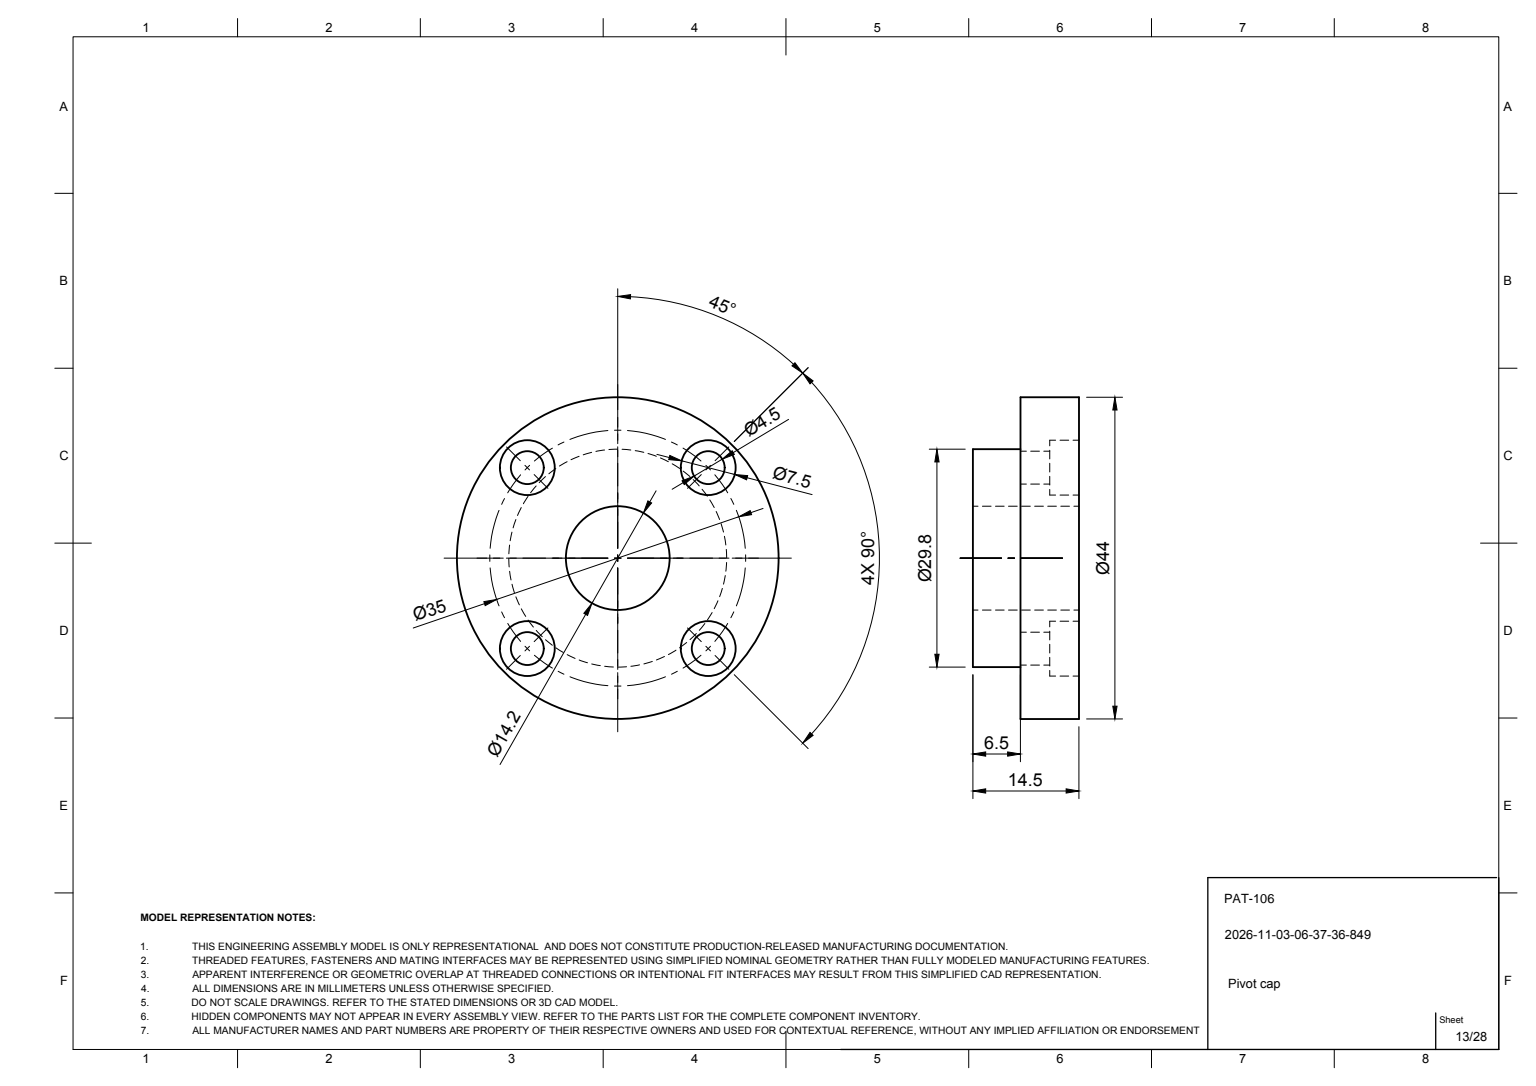
ISO-10303-21;
HEADER;
/* Generated by software containing ST-Developer
 * from STEP Tools, Inc. (www.steptools.com) 
 */

FILE_DESCRIPTION(
/* description */ ('Torsion-spring ratchet demonstrator'),
/* implementation_level */ '2;1');

FILE_NAME(
/* name */ 'Pivot cap.step',
/* time_stamp */ '2026-10-29T17:29:17-07:00',
/* author */ (''),
/* organization */ (''),
/* preprocessor_version */ 'ST-DEVELOPER v20.2',
/* originating_system */ 'Autodesk Translation Framework v15.17.0.0',
/* authorisation */ '');

FILE_SCHEMA (('AUTOMOTIVE_DESIGN { 1 0 10303 214 3 1 1 }'));
ENDSEC;

DATA;
#10=MECHANICAL_DESIGN_GEOMETRIC_PRESENTATION_REPRESENTATION('',(#291),#11258);
#243=SHAPE_REPRESENTATION_RELATIONSHIP('SRR','None',#11369,#267);
#267=ADVANCED_BREP_SHAPE_REPRESENTATION('',(#323),#11239);
#291=STYLED_ITEM('',(#11570),#323);
#323=MANIFOLD_SOLID_BREP('Body1',#5162);
#394=FACE_BOUND('',#1065,.T.);
#395=FACE_BOUND('',#1068,.T.);
#396=FACE_BOUND('',#1071,.T.);
#397=FACE_BOUND('',#1074,.T.);
#398=FACE_BOUND('',#1081,.T.);
#399=FACE_BOUND('',#1085,.T.);
#400=FACE_BOUND('',#1086,.T.);
#401=FACE_BOUND('',#1087,.T.);
#402=FACE_BOUND('',#1088,.T.);
#403=FACE_BOUND('',#1089,.T.);
#404=FACE_BOUND('',#1091,.T.);
#405=FACE_BOUND('',#1092,.T.);
#406=FACE_BOUND('',#1093,.T.);
#407=FACE_BOUND('',#1094,.T.);
#408=FACE_BOUND('',#1095,.T.);
#482=PLANE('',#5643);
#483=PLANE('',#5648);
#484=PLANE('',#5653);
#485=PLANE('',#5658);
#486=PLANE('',#5671);
#487=PLANE('',#5678);
#488=PLANE('',#5679);
#709=FACE_OUTER_BOUND('',#1063,.T.);
#710=FACE_OUTER_BOUND('',#1064,.T.);
#711=FACE_OUTER_BOUND('',#1066,.T.);
#712=FACE_OUTER_BOUND('',#1067,.T.);
#713=FACE_OUTER_BOUND('',#1069,.T.);
#714=FACE_OUTER_BOUND('',#1070,.T.);
#715=FACE_OUTER_BOUND('',#1072,.T.);
#716=FACE_OUTER_BOUND('',#1073,.T.);
#717=FACE_OUTER_BOUND('',#1075,.T.);
#718=FACE_OUTER_BOUND('',#1076,.T.);
#719=FACE_OUTER_BOUND('',#1077,.T.);
#720=FACE_OUTER_BOUND('',#1078,.T.);
#721=FACE_OUTER_BOUND('',#1079,.T.);
#722=FACE_OUTER_BOUND('',#1080,.T.);
#723=FACE_OUTER_BOUND('',#1082,.T.);
#724=FACE_OUTER_BOUND('',#1083,.T.);
#725=FACE_OUTER_BOUND('',#1084,.T.);
#726=FACE_OUTER_BOUND('',#1090,.T.);
#1063=EDGE_LOOP('',(#3796,#3797,#3798,#3799));
#1064=EDGE_LOOP('',(#3800));
#1065=EDGE_LOOP('',(#3801));
#1066=EDGE_LOOP('',(#3802,#3803,#3804,#3805));
#1067=EDGE_LOOP('',(#3806));
#1068=EDGE_LOOP('',(#3807));
#1069=EDGE_LOOP('',(#3808,#3809,#3810,#3811));
#1070=EDGE_LOOP('',(#3812));
#1071=EDGE_LOOP('',(#3813));
#1072=EDGE_LOOP('',(#3814,#3815,#3816,#3817));
#1073=EDGE_LOOP('',(#3818));
#1074=EDGE_LOOP('',(#3819));
#1075=EDGE_LOOP('',(#3820,#3821,#3822,#3823));
#1076=EDGE_LOOP('',(#3824,#3825,#3826,#3827));
#1077=EDGE_LOOP('',(#3828,#3829,#3830,#3831));
#1078=EDGE_LOOP('',(#3832,#3833,#3834,#3835));
#1079=EDGE_LOOP('',(#3836,#3837,#3838,#3839));
#1080=EDGE_LOOP('',(#3840));
#1081=EDGE_LOOP('',(#3841));
#1082=EDGE_LOOP('',(#3842,#3843,#3844,#3845));
#1083=EDGE_LOOP('',(#3846,#3847,#3848,#3849));
#1084=EDGE_LOOP('',(#3850));
#1085=EDGE_LOOP('',(#3851));
#1086=EDGE_LOOP('',(#3852));
#1087=EDGE_LOOP('',(#3853));
#1088=EDGE_LOOP('',(#3854));
#1089=EDGE_LOOP('',(#3855));
#1090=EDGE_LOOP('',(#3856));
#1091=EDGE_LOOP('',(#3857));
#1092=EDGE_LOOP('',(#3858));
#1093=EDGE_LOOP('',(#3859));
#1094=EDGE_LOOP('',(#3860));
#1095=EDGE_LOOP('',(#3861));
#1408=LINE('',#8139,#1791);
#1409=LINE('',#8148,#1792);
#1410=LINE('',#8157,#1793);
#1411=LINE('',#8166,#1794);
#1412=LINE('',#8174,#1795);
#1413=LINE('',#8178,#1796);
#1414=LINE('',#8182,#1797);
#1415=LINE('',#8186,#1798);
#1416=LINE('',#8191,#1799);
#1417=LINE('',#8199,#1800);
#1418=LINE('',#8204,#1801);
#1791=VECTOR('',#6527,0.375);
#1792=VECTOR('',#6538,0.375);
#1793=VECTOR('',#6549,0.375);
#1794=VECTOR('',#6560,0.375);
#1795=VECTOR('',#6571,0.225);
#1796=VECTOR('',#6576,0.225);
#1797=VECTOR('',#6581,0.225);
#1798=VECTOR('',#6586,0.225);
#1799=VECTOR('',#6591,1.49);
#1800=VECTOR('',#6602,0.71);
#1801=VECTOR('',#6607,2.2);
#2181=CIRCLE('',#5641,0.375);
#2182=CIRCLE('',#5642,0.375);
#2183=CIRCLE('',#5644,0.225);
#2184=CIRCLE('',#5646,0.375);
#2185=CIRCLE('',#5647,0.375);
#2186=CIRCLE('',#5649,0.225);
#2187=CIRCLE('',#5651,0.375);
#2188=CIRCLE('',#5652,0.375);
#2189=CIRCLE('',#5654,0.225);
#2190=CIRCLE('',#5656,0.375);
#2191=CIRCLE('',#5657,0.375);
#2192=CIRCLE('',#5659,0.225);
#2193=CIRCLE('',#5661,0.225);
#2194=CIRCLE('',#5663,0.225);
#2195=CIRCLE('',#5665,0.225);
#2196=CIRCLE('',#5667,0.225);
#2197=CIRCLE('',#5669,1.49);
#2198=CIRCLE('',#5670,1.49);
#2199=CIRCLE('',#5672,0.71);
#2200=CIRCLE('',#5674,0.71);
#2201=CIRCLE('',#5676,2.2);
#2202=CIRCLE('',#5677,2.2);
#2453=VERTEX_POINT('',#8136);
#2454=VERTEX_POINT('',#8138);
#2455=VERTEX_POINT('',#8142);
#2456=VERTEX_POINT('',#8145);
#2457=VERTEX_POINT('',#8147);
#2458=VERTEX_POINT('',#8151);
#2459=VERTEX_POINT('',#8154);
#2460=VERTEX_POINT('',#8156);
#2461=VERTEX_POINT('',#8160);
#2462=VERTEX_POINT('',#8163);
#2463=VERTEX_POINT('',#8165);
#2464=VERTEX_POINT('',#8169);
#2465=VERTEX_POINT('',#8172);
#2466=VERTEX_POINT('',#8176);
#2467=VERTEX_POINT('',#8180);
#2468=VERTEX_POINT('',#8184);
#2469=VERTEX_POINT('',#8188);
#2470=VERTEX_POINT('',#8190);
#2471=VERTEX_POINT('',#8194);
#2472=VERTEX_POINT('',#8197);
#2473=VERTEX_POINT('',#8201);
#2474=VERTEX_POINT('',#8203);
#2958=EDGE_CURVE('',#2453,#2453,#2181,.T.);
#2959=EDGE_CURVE('',#2453,#2454,#1408,.T.);
#2960=EDGE_CURVE('',#2454,#2454,#2182,.T.);
#2961=EDGE_CURVE('',#2455,#2455,#2183,.T.);
#2962=EDGE_CURVE('',#2456,#2456,#2184,.T.);
#2963=EDGE_CURVE('',#2456,#2457,#1409,.T.);
#2964=EDGE_CURVE('',#2457,#2457,#2185,.T.);
#2965=EDGE_CURVE('',#2458,#2458,#2186,.T.);
#2966=EDGE_CURVE('',#2459,#2459,#2187,.T.);
#2967=EDGE_CURVE('',#2459,#2460,#1410,.T.);
#2968=EDGE_CURVE('',#2460,#2460,#2188,.T.);
#2969=EDGE_CURVE('',#2461,#2461,#2189,.T.);
#2970=EDGE_CURVE('',#2462,#2462,#2190,.T.);
#2971=EDGE_CURVE('',#2462,#2463,#1411,.T.);
#2972=EDGE_CURVE('',#2463,#2463,#2191,.T.);
#2973=EDGE_CURVE('',#2464,#2464,#2192,.T.);
#2974=EDGE_CURVE('',#2465,#2465,#2193,.T.);
#2975=EDGE_CURVE('',#2465,#2455,#1412,.T.);
#2976=EDGE_CURVE('',#2466,#2466,#2194,.T.);
#2977=EDGE_CURVE('',#2466,#2458,#1413,.T.);
#2978=EDGE_CURVE('',#2467,#2467,#2195,.T.);
#2979=EDGE_CURVE('',#2467,#2461,#1414,.T.);
#2980=EDGE_CURVE('',#2468,#2468,#2196,.T.);
#2981=EDGE_CURVE('',#2468,#2464,#1415,.T.);
#2982=EDGE_CURVE('',#2469,#2469,#2197,.T.);
#2983=EDGE_CURVE('',#2469,#2470,#1416,.T.);
#2984=EDGE_CURVE('',#2470,#2470,#2198,.T.);
#2985=EDGE_CURVE('',#2471,#2471,#2199,.T.);
#2986=EDGE_CURVE('',#2472,#2472,#2200,.T.);
#2987=EDGE_CURVE('',#2472,#2471,#1417,.T.);
#2988=EDGE_CURVE('',#2473,#2473,#2201,.T.);
#2989=EDGE_CURVE('',#2473,#2474,#1418,.T.);
#2990=EDGE_CURVE('',#2474,#2474,#2202,.T.);
#3796=ORIENTED_EDGE('',*,*,#2958,.F.);
#3797=ORIENTED_EDGE('',*,*,#2959,.T.);
#3798=ORIENTED_EDGE('',*,*,#2960,.F.);
#3799=ORIENTED_EDGE('',*,*,#2959,.F.);
#3800=ORIENTED_EDGE('',*,*,#2958,.T.);
#3801=ORIENTED_EDGE('',*,*,#2961,.F.);
#3802=ORIENTED_EDGE('',*,*,#2962,.F.);
#3803=ORIENTED_EDGE('',*,*,#2963,.T.);
#3804=ORIENTED_EDGE('',*,*,#2964,.F.);
#3805=ORIENTED_EDGE('',*,*,#2963,.F.);
#3806=ORIENTED_EDGE('',*,*,#2962,.T.);
#3807=ORIENTED_EDGE('',*,*,#2965,.F.);
#3808=ORIENTED_EDGE('',*,*,#2966,.F.);
#3809=ORIENTED_EDGE('',*,*,#2967,.T.);
#3810=ORIENTED_EDGE('',*,*,#2968,.F.);
#3811=ORIENTED_EDGE('',*,*,#2967,.F.);
#3812=ORIENTED_EDGE('',*,*,#2966,.T.);
#3813=ORIENTED_EDGE('',*,*,#2969,.F.);
#3814=ORIENTED_EDGE('',*,*,#2970,.F.);
#3815=ORIENTED_EDGE('',*,*,#2971,.T.);
#3816=ORIENTED_EDGE('',*,*,#2972,.F.);
#3817=ORIENTED_EDGE('',*,*,#2971,.F.);
#3818=ORIENTED_EDGE('',*,*,#2970,.T.);
#3819=ORIENTED_EDGE('',*,*,#2973,.F.);
#3820=ORIENTED_EDGE('',*,*,#2974,.F.);
#3821=ORIENTED_EDGE('',*,*,#2975,.T.);
#3822=ORIENTED_EDGE('',*,*,#2961,.T.);
#3823=ORIENTED_EDGE('',*,*,#2975,.F.);
#3824=ORIENTED_EDGE('',*,*,#2976,.F.);
#3825=ORIENTED_EDGE('',*,*,#2977,.T.);
#3826=ORIENTED_EDGE('',*,*,#2965,.T.);
#3827=ORIENTED_EDGE('',*,*,#2977,.F.);
#3828=ORIENTED_EDGE('',*,*,#2978,.F.);
#3829=ORIENTED_EDGE('',*,*,#2979,.T.);
#3830=ORIENTED_EDGE('',*,*,#2969,.T.);
#3831=ORIENTED_EDGE('',*,*,#2979,.F.);
#3832=ORIENTED_EDGE('',*,*,#2980,.F.);
#3833=ORIENTED_EDGE('',*,*,#2981,.T.);
#3834=ORIENTED_EDGE('',*,*,#2973,.T.);
#3835=ORIENTED_EDGE('',*,*,#2981,.F.);
#3836=ORIENTED_EDGE('',*,*,#2982,.F.);
#3837=ORIENTED_EDGE('',*,*,#2983,.T.);
#3838=ORIENTED_EDGE('',*,*,#2984,.T.);
#3839=ORIENTED_EDGE('',*,*,#2983,.F.);
#3840=ORIENTED_EDGE('',*,*,#2984,.F.);
#3841=ORIENTED_EDGE('',*,*,#2985,.F.);
#3842=ORIENTED_EDGE('',*,*,#2986,.F.);
#3843=ORIENTED_EDGE('',*,*,#2987,.T.);
#3844=ORIENTED_EDGE('',*,*,#2985,.T.);
#3845=ORIENTED_EDGE('',*,*,#2987,.F.);
#3846=ORIENTED_EDGE('',*,*,#2988,.F.);
#3847=ORIENTED_EDGE('',*,*,#2989,.T.);
#3848=ORIENTED_EDGE('',*,*,#2990,.T.);
#3849=ORIENTED_EDGE('',*,*,#2989,.F.);
#3850=ORIENTED_EDGE('',*,*,#2988,.T.);
#3851=ORIENTED_EDGE('',*,*,#2986,.T.);
#3852=ORIENTED_EDGE('',*,*,#2972,.T.);
#3853=ORIENTED_EDGE('',*,*,#2968,.T.);
#3854=ORIENTED_EDGE('',*,*,#2964,.T.);
#3855=ORIENTED_EDGE('',*,*,#2960,.T.);
#3856=ORIENTED_EDGE('',*,*,#2990,.F.);
#3857=ORIENTED_EDGE('',*,*,#2982,.T.);
#3858=ORIENTED_EDGE('',*,*,#2980,.T.);
#3859=ORIENTED_EDGE('',*,*,#2978,.T.);
#3860=ORIENTED_EDGE('',*,*,#2976,.T.);
#3861=ORIENTED_EDGE('',*,*,#2974,.T.);
#4805=CYLINDRICAL_SURFACE('',#5640,0.375);
#4806=CYLINDRICAL_SURFACE('',#5645,0.375);
#4807=CYLINDRICAL_SURFACE('',#5650,0.375);
#4808=CYLINDRICAL_SURFACE('',#5655,0.375);
#4809=CYLINDRICAL_SURFACE('',#5660,0.225);
#4810=CYLINDRICAL_SURFACE('',#5662,0.225);
#4811=CYLINDRICAL_SURFACE('',#5664,0.225);
#4812=CYLINDRICAL_SURFACE('',#5666,0.225);
#4813=CYLINDRICAL_SURFACE('',#5668,1.49);
#4814=CYLINDRICAL_SURFACE('',#5673,0.71);
#4815=CYLINDRICAL_SURFACE('',#5675,2.2);
#4935=ADVANCED_FACE('',(#709),#4805,.F.);
#4936=ADVANCED_FACE('',(#710,#394),#482,.T.);
#4937=ADVANCED_FACE('',(#711),#4806,.F.);
#4938=ADVANCED_FACE('',(#712,#395),#483,.T.);
#4939=ADVANCED_FACE('',(#713),#4807,.F.);
#4940=ADVANCED_FACE('',(#714,#396),#484,.T.);
#4941=ADVANCED_FACE('',(#715),#4808,.F.);
#4942=ADVANCED_FACE('',(#716,#397),#485,.T.);
#4943=ADVANCED_FACE('',(#717),#4809,.F.);
#4944=ADVANCED_FACE('',(#718),#4810,.F.);
#4945=ADVANCED_FACE('',(#719),#4811,.F.);
#4946=ADVANCED_FACE('',(#720),#4812,.F.);
#4947=ADVANCED_FACE('',(#721),#4813,.T.);
#4948=ADVANCED_FACE('',(#722,#398),#486,.F.);
#4949=ADVANCED_FACE('',(#723),#4814,.F.);
#4950=ADVANCED_FACE('',(#724),#4815,.T.);
#4951=ADVANCED_FACE('',(#725,#399,#400,#401,#402,#403),#487,.T.);
#4952=ADVANCED_FACE('',(#726,#404,#405,#406,#407,#408),#488,.F.);
#5162=CLOSED_SHELL('',(#4935,#4936,#4937,#4938,#4939,#4940,#4941,#4942,
#4943,#4944,#4945,#4946,#4947,#4948,#4949,#4950,#4951,#4952));
#5639=AXIS2_PLACEMENT_3D('',#8134,#6521,#6522);
#5640=AXIS2_PLACEMENT_3D('',#8135,#6523,#6524);
#5641=AXIS2_PLACEMENT_3D('',#8137,#6525,#6526);
#5642=AXIS2_PLACEMENT_3D('',#8140,#6528,#6529);
#5643=AXIS2_PLACEMENT_3D('',#8141,#6530,#6531);
#5644=AXIS2_PLACEMENT_3D('',#8143,#6532,#6533);
#5645=AXIS2_PLACEMENT_3D('',#8144,#6534,#6535);
#5646=AXIS2_PLACEMENT_3D('',#8146,#6536,#6537);
#5647=AXIS2_PLACEMENT_3D('',#8149,#6539,#6540);
#5648=AXIS2_PLACEMENT_3D('',#8150,#6541,#6542);
#5649=AXIS2_PLACEMENT_3D('',#8152,#6543,#6544);
#5650=AXIS2_PLACEMENT_3D('',#8153,#6545,#6546);
#5651=AXIS2_PLACEMENT_3D('',#8155,#6547,#6548);
#5652=AXIS2_PLACEMENT_3D('',#8158,#6550,#6551);
#5653=AXIS2_PLACEMENT_3D('',#8159,#6552,#6553);
#5654=AXIS2_PLACEMENT_3D('',#8161,#6554,#6555);
#5655=AXIS2_PLACEMENT_3D('',#8162,#6556,#6557);
#5656=AXIS2_PLACEMENT_3D('',#8164,#6558,#6559);
#5657=AXIS2_PLACEMENT_3D('',#8167,#6561,#6562);
#5658=AXIS2_PLACEMENT_3D('',#8168,#6563,#6564);
#5659=AXIS2_PLACEMENT_3D('',#8170,#6565,#6566);
#5660=AXIS2_PLACEMENT_3D('',#8171,#6567,#6568);
#5661=AXIS2_PLACEMENT_3D('',#8173,#6569,#6570);
#5662=AXIS2_PLACEMENT_3D('',#8175,#6572,#6573);
#5663=AXIS2_PLACEMENT_3D('',#8177,#6574,#6575);
#5664=AXIS2_PLACEMENT_3D('',#8179,#6577,#6578);
#5665=AXIS2_PLACEMENT_3D('',#8181,#6579,#6580);
#5666=AXIS2_PLACEMENT_3D('',#8183,#6582,#6583);
#5667=AXIS2_PLACEMENT_3D('',#8185,#6584,#6585);
#5668=AXIS2_PLACEMENT_3D('',#8187,#6587,#6588);
#5669=AXIS2_PLACEMENT_3D('',#8189,#6589,#6590);
#5670=AXIS2_PLACEMENT_3D('',#8192,#6592,#6593);
#5671=AXIS2_PLACEMENT_3D('',#8193,#6594,#6595);
#5672=AXIS2_PLACEMENT_3D('',#8195,#6596,#6597);
#5673=AXIS2_PLACEMENT_3D('',#8196,#6598,#6599);
#5674=AXIS2_PLACEMENT_3D('',#8198,#6600,#6601);
#5675=AXIS2_PLACEMENT_3D('',#8200,#6603,#6604);
#5676=AXIS2_PLACEMENT_3D('',#8202,#6605,#6606);
#5677=AXIS2_PLACEMENT_3D('',#8205,#6608,#6609);
#5678=AXIS2_PLACEMENT_3D('',#8206,#6610,#6611);
#5679=AXIS2_PLACEMENT_3D('',#8207,#6612,#6613);
#6521=DIRECTION('axis',(0.,0.,1.));
#6522=DIRECTION('refdir',(1.,0.,0.));
#6523=DIRECTION('center_axis',(0.,0.,1.));
#6524=DIRECTION('ref_axis',(1.,0.,0.));
#6525=DIRECTION('center_axis',(0.,0.,1.));
#6526=DIRECTION('ref_axis',(1.,0.,0.));
#6527=DIRECTION('',(0.,0.,1.));
#6528=DIRECTION('center_axis',(0.,0.,-1.));
#6529=DIRECTION('ref_axis',(1.,0.,0.));
#6530=DIRECTION('center_axis',(0.,0.,1.));
#6531=DIRECTION('ref_axis',(1.,0.,0.));
#6532=DIRECTION('center_axis',(0.,0.,1.));
#6533=DIRECTION('ref_axis',(1.,0.,0.));
#6534=DIRECTION('center_axis',(0.,0.,1.));
#6535=DIRECTION('ref_axis',(1.,0.,0.));
#6536=DIRECTION('center_axis',(0.,0.,1.));
#6537=DIRECTION('ref_axis',(1.,0.,0.));
#6538=DIRECTION('',(0.,0.,1.));
#6539=DIRECTION('center_axis',(0.,0.,-1.));
#6540=DIRECTION('ref_axis',(1.,0.,0.));
#6541=DIRECTION('center_axis',(0.,0.,1.));
#6542=DIRECTION('ref_axis',(1.,0.,0.));
#6543=DIRECTION('center_axis',(0.,0.,1.));
#6544=DIRECTION('ref_axis',(1.,0.,0.));
#6545=DIRECTION('center_axis',(0.,0.,1.));
#6546=DIRECTION('ref_axis',(1.,0.,0.));
#6547=DIRECTION('center_axis',(0.,0.,1.));
#6548=DIRECTION('ref_axis',(1.,0.,0.));
#6549=DIRECTION('',(0.,0.,1.));
#6550=DIRECTION('center_axis',(0.,0.,-1.));
#6551=DIRECTION('ref_axis',(1.,0.,0.));
#6552=DIRECTION('center_axis',(0.,0.,1.));
#6553=DIRECTION('ref_axis',(1.,0.,0.));
#6554=DIRECTION('center_axis',(0.,0.,1.));
#6555=DIRECTION('ref_axis',(1.,0.,0.));
#6556=DIRECTION('center_axis',(0.,0.,1.));
#6557=DIRECTION('ref_axis',(1.,0.,0.));
#6558=DIRECTION('center_axis',(0.,0.,1.));
#6559=DIRECTION('ref_axis',(1.,0.,0.));
#6560=DIRECTION('',(0.,0.,1.));
#6561=DIRECTION('center_axis',(0.,0.,-1.));
#6562=DIRECTION('ref_axis',(1.,0.,0.));
#6563=DIRECTION('center_axis',(0.,0.,1.));
#6564=DIRECTION('ref_axis',(1.,0.,0.));
#6565=DIRECTION('center_axis',(0.,0.,1.));
#6566=DIRECTION('ref_axis',(1.,0.,0.));
#6567=DIRECTION('center_axis',(0.,0.,1.));
#6568=DIRECTION('ref_axis',(1.,0.,0.));
#6569=DIRECTION('center_axis',(0.,0.,1.));
#6570=DIRECTION('ref_axis',(1.,0.,0.));
#6571=DIRECTION('',(0.,0.,1.));
#6572=DIRECTION('center_axis',(0.,0.,1.));
#6573=DIRECTION('ref_axis',(1.,0.,0.));
#6574=DIRECTION('center_axis',(0.,0.,1.));
#6575=DIRECTION('ref_axis',(1.,0.,0.));
#6576=DIRECTION('',(0.,0.,1.));
#6577=DIRECTION('center_axis',(0.,0.,1.));
#6578=DIRECTION('ref_axis',(1.,0.,0.));
#6579=DIRECTION('center_axis',(0.,0.,1.));
#6580=DIRECTION('ref_axis',(1.,0.,0.));
#6581=DIRECTION('',(0.,0.,1.));
#6582=DIRECTION('center_axis',(0.,0.,1.));
#6583=DIRECTION('ref_axis',(1.,0.,0.));
#6584=DIRECTION('center_axis',(0.,0.,1.));
#6585=DIRECTION('ref_axis',(1.,0.,0.));
#6586=DIRECTION('',(0.,0.,1.));
#6587=DIRECTION('center_axis',(0.,0.,1.));
#6588=DIRECTION('ref_axis',(1.,0.,0.));
#6589=DIRECTION('center_axis',(0.,0.,1.));
#6590=DIRECTION('ref_axis',(1.,0.,0.));
#6591=DIRECTION('',(0.,0.,-1.));
#6592=DIRECTION('center_axis',(0.,0.,1.));
#6593=DIRECTION('ref_axis',(1.,0.,0.));
#6594=DIRECTION('center_axis',(0.,0.,1.));
#6595=DIRECTION('ref_axis',(1.,0.,0.));
#6596=DIRECTION('center_axis',(0.,0.,-1.));
#6597=DIRECTION('ref_axis',(1.,0.,0.));
#6598=DIRECTION('center_axis',(0.,0.,1.));
#6599=DIRECTION('ref_axis',(1.,0.,0.));
#6600=DIRECTION('center_axis',(0.,0.,-1.));
#6601=DIRECTION('ref_axis',(1.,0.,0.));
#6602=DIRECTION('',(0.,0.,-1.));
#6603=DIRECTION('center_axis',(0.,0.,1.));
#6604=DIRECTION('ref_axis',(1.,0.,0.));
#6605=DIRECTION('center_axis',(0.,0.,1.));
#6606=DIRECTION('ref_axis',(1.,0.,0.));
#6607=DIRECTION('',(0.,0.,-1.));
#6608=DIRECTION('center_axis',(0.,0.,1.));
#6609=DIRECTION('ref_axis',(1.,0.,0.));
#6610=DIRECTION('center_axis',(0.,0.,1.));
#6611=DIRECTION('ref_axis',(1.,0.,0.));
#6612=DIRECTION('center_axis',(0.,0.,1.));
#6613=DIRECTION('ref_axis',(1.,0.,0.));
#8134=CARTESIAN_POINT('',(0.,0.,0.));
#8135=CARTESIAN_POINT('Origin',(-1.23743686707646,-1.23743686707646,4.));
#8136=CARTESIAN_POINT('',(-1.61243686707646,-1.23743686707646,4.));
#8137=CARTESIAN_POINT('Origin',(-1.23743686707646,-1.23743686707646,4.));
#8138=CARTESIAN_POINT('',(-1.61243686707646,-1.23743686707646,4.4));
#8139=CARTESIAN_POINT('',(-1.61243686707646,-1.23743686707646,4.));
#8140=CARTESIAN_POINT('Origin',(-1.23743686707646,-1.23743686707646,4.4));
#8141=CARTESIAN_POINT('Origin',(-1.23743686707646,-1.23743686707646,4.));
#8142=CARTESIAN_POINT('',(-1.46243686707646,-1.23743686707646,4.));
#8143=CARTESIAN_POINT('Origin',(-1.23743686707646,-1.23743686707646,4.));
#8144=CARTESIAN_POINT('Origin',(-1.23743686707646,1.23743686707646,4.));
#8145=CARTESIAN_POINT('',(-1.61243686707646,1.23743686707646,4.));
#8146=CARTESIAN_POINT('Origin',(-1.23743686707646,1.23743686707646,4.));
#8147=CARTESIAN_POINT('',(-1.61243686707646,1.23743686707646,4.4));
#8148=CARTESIAN_POINT('',(-1.61243686707646,1.23743686707646,4.));
#8149=CARTESIAN_POINT('Origin',(-1.23743686707646,1.23743686707646,4.4));
#8150=CARTESIAN_POINT('Origin',(-1.23743686707646,1.23743686707646,4.));
#8151=CARTESIAN_POINT('',(-1.46243686707646,1.23743686707646,4.));
#8152=CARTESIAN_POINT('Origin',(-1.23743686707646,1.23743686707646,4.));
#8153=CARTESIAN_POINT('Origin',(1.23743686707646,1.23743686707646,4.));
#8154=CARTESIAN_POINT('',(0.862436867076458,1.23743686707646,4.));
#8155=CARTESIAN_POINT('Origin',(1.23743686707646,1.23743686707646,4.));
#8156=CARTESIAN_POINT('',(0.862436867076458,1.23743686707646,4.4));
#8157=CARTESIAN_POINT('',(0.862436867076458,1.23743686707646,4.));
#8158=CARTESIAN_POINT('Origin',(1.23743686707646,1.23743686707646,4.4));
#8159=CARTESIAN_POINT('Origin',(1.23743686707646,1.23743686707646,4.));
#8160=CARTESIAN_POINT('',(1.01243686707646,1.23743686707646,4.));
#8161=CARTESIAN_POINT('Origin',(1.23743686707646,1.23743686707646,4.));
#8162=CARTESIAN_POINT('Origin',(1.23743686707646,-1.23743686707646,4.));
#8163=CARTESIAN_POINT('',(0.862436867076458,-1.23743686707646,4.));
#8164=CARTESIAN_POINT('Origin',(1.23743686707646,-1.23743686707646,4.));
#8165=CARTESIAN_POINT('',(0.862436867076458,-1.23743686707646,4.4));
#8166=CARTESIAN_POINT('',(0.862436867076458,-1.23743686707646,4.));
#8167=CARTESIAN_POINT('Origin',(1.23743686707646,-1.23743686707646,4.4));
#8168=CARTESIAN_POINT('Origin',(1.23743686707646,-1.23743686707646,4.));
#8169=CARTESIAN_POINT('',(1.01243686707646,-1.23743686707646,4.));
#8170=CARTESIAN_POINT('Origin',(1.23743686707646,-1.23743686707646,4.));
#8171=CARTESIAN_POINT('Origin',(-1.23743686707646,-1.23743686707646,3.5));
#8172=CARTESIAN_POINT('',(-1.46243686707646,-1.23743686707646,3.6));
#8173=CARTESIAN_POINT('Origin',(-1.23743686707646,-1.23743686707646,3.6));
#8174=CARTESIAN_POINT('',(-1.46243686707646,-1.23743686707646,3.5));
#8175=CARTESIAN_POINT('Origin',(-1.23743686707646,1.23743686707646,3.5));
#8176=CARTESIAN_POINT('',(-1.46243686707646,1.23743686707646,3.6));
#8177=CARTESIAN_POINT('Origin',(-1.23743686707646,1.23743686707646,3.6));
#8178=CARTESIAN_POINT('',(-1.46243686707646,1.23743686707646,3.5));
#8179=CARTESIAN_POINT('Origin',(1.23743686707646,1.23743686707646,3.5));
#8180=CARTESIAN_POINT('',(1.01243686707646,1.23743686707646,3.6));
#8181=CARTESIAN_POINT('Origin',(1.23743686707646,1.23743686707646,3.6));
#8182=CARTESIAN_POINT('',(1.01243686707646,1.23743686707646,3.5));
#8183=CARTESIAN_POINT('Origin',(1.23743686707646,-1.23743686707646,3.5));
#8184=CARTESIAN_POINT('',(1.01243686707646,-1.23743686707646,3.6));
#8185=CARTESIAN_POINT('Origin',(1.23743686707646,-1.23743686707646,3.6));
#8186=CARTESIAN_POINT('',(1.01243686707646,-1.23743686707646,3.5));
#8187=CARTESIAN_POINT('Origin',(0.,0.,2.95));
#8188=CARTESIAN_POINT('',(-1.49,-1.82472373072956E-16,3.6));
#8189=CARTESIAN_POINT('Origin',(0.,0.,3.6));
#8190=CARTESIAN_POINT('',(-1.49,-1.82472373072956E-16,2.95));
#8191=CARTESIAN_POINT('',(-1.49,-1.82472373072956E-16,2.95));
#8192=CARTESIAN_POINT('Origin',(0.,0.,2.95));
#8193=CARTESIAN_POINT('Origin',(0.,0.,2.95));
#8194=CARTESIAN_POINT('',(-0.71,-8.69499227394621E-17,2.95));
#8195=CARTESIAN_POINT('Origin',(0.,0.,2.95));
#8196=CARTESIAN_POINT('Origin',(0.,0.,3.6));
#8197=CARTESIAN_POINT('',(-0.71,-8.69499227394621E-17,4.4));
#8198=CARTESIAN_POINT('Origin',(0.,0.,4.4));
#8199=CARTESIAN_POINT('',(-0.71,-8.69499227394621E-17,3.6));
#8200=CARTESIAN_POINT('Origin',(0.,0.,3.6));
#8201=CARTESIAN_POINT('',(-2.2,-2.69422295812418E-16,4.4));
#8202=CARTESIAN_POINT('Origin',(0.,0.,4.4));
#8203=CARTESIAN_POINT('',(-2.2,-2.69422295812418E-16,3.6));
#8204=CARTESIAN_POINT('',(-2.2,-2.69422295812418E-16,3.6));
#8205=CARTESIAN_POINT('Origin',(0.,0.,3.6));
#8206=CARTESIAN_POINT('Origin',(0.,0.,4.4));
#8207=CARTESIAN_POINT('Origin',(0.,0.,3.6));
#11209=UNCERTAINTY_MEASURE_WITH_UNIT(LENGTH_MEASURE(0.001),#11259,
'DISTANCE_ACCURACY_VALUE',
'Maximum model space distance between geometric entities at asserted c
onnectivities');
#11228=UNCERTAINTY_MEASURE_WITH_UNIT(LENGTH_MEASURE(0.001),#11259,
'DISTANCE_ACCURACY_VALUE',
'Maximum model space distance between geometric entities at asserted c
onnectivities');
#11239=(
GEOMETRIC_REPRESENTATION_CONTEXT(3)
GLOBAL_UNCERTAINTY_ASSIGNED_CONTEXT((#11209))
GLOBAL_UNIT_ASSIGNED_CONTEXT((#11259,#11261,#11262))
REPRESENTATION_CONTEXT('','3D')
);
#11258=(
GEOMETRIC_REPRESENTATION_CONTEXT(3)
GLOBAL_UNCERTAINTY_ASSIGNED_CONTEXT((#11228))
GLOBAL_UNIT_ASSIGNED_CONTEXT((#11259,#11261,#11262))
REPRESENTATION_CONTEXT('','3D')
);
#11259=(
LENGTH_UNIT()
NAMED_UNIT(*)
SI_UNIT(.CENTI.,.METRE.)
);
#11261=(
NAMED_UNIT(*)
PLANE_ANGLE_UNIT()
SI_UNIT($,.RADIAN.)
);
#11262=(
NAMED_UNIT(*)
SI_UNIT($,.STERADIAN.)
SOLID_ANGLE_UNIT()
);
#11273=SHAPE_DEFINITION_REPRESENTATION(#11302,#11369);
#11302=PRODUCT_DEFINITION_SHAPE('',$,#11399);
#11369=SHAPE_REPRESENTATION('',(#5639),#11239);
#11388=PRODUCT_DEFINITION_CONTEXT('part definition',#11477,'design');
#11399=PRODUCT_DEFINITION('Pivot cap','Pivot cap',#11428,#11388);
#11428=PRODUCT_DEFINITION_FORMATION('',$,#11489);
#11477=APPLICATION_CONTEXT(
'Core Data for Automotive Mechanical Design Process');
#11478=PRODUCT_CONTEXT('part definition',#11477,'mechanical');
#11489=PRODUCT('Pivot cap','Pivot cap','Pivot cap',(#11478));
#11564=COLOUR_RGB('Light Blue',0.38,0.62,0.78);
#11565=FILL_AREA_STYLE_COLOUR('',#11564);
#11566=FILL_AREA_STYLE('',(#11565));
#11567=SURFACE_STYLE_FILL_AREA(#11566);
#11568=SURFACE_SIDE_STYLE('',(#11567));
#11569=SURFACE_STYLE_USAGE(.BOTH.,#11568);
#11570=PRESENTATION_STYLE_ASSIGNMENT((#11569));
ENDSEC;
END-ISO-10303-21;
